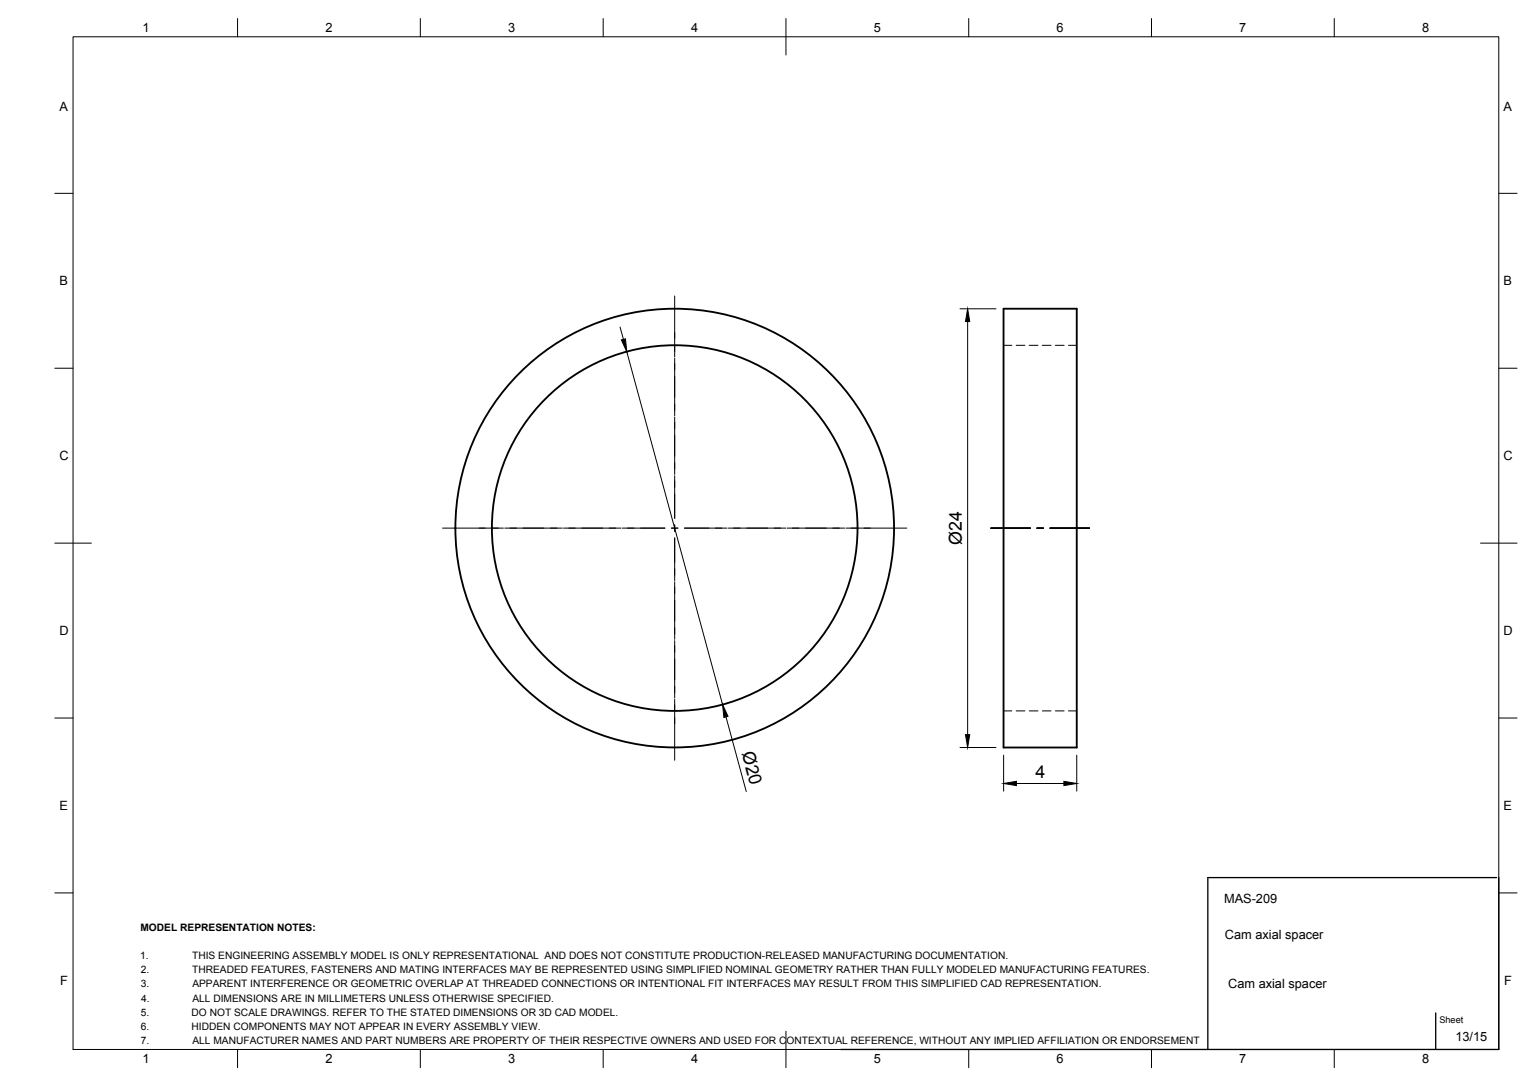
ISO-10303-21;
HEADER;
/* Generated by software containing ST-Developer
 * from STEP Tools, Inc. (www.steptools.com) 
 */

FILE_DESCRIPTION(
/* description */ ('Independent bearing-supported roller-ramp one-way clutch. Six logarit
hmic ramps with plain solid rollers, sprung guided plungers, native Co
il variants, removable shared keepers, rounded parallel key, shaft wit
h complete retaining lips, bronze journal/thrust support and bolted co
vers. Native rotor, roller planar/spin and plunger joints permit manua
l geometric engaged/released inspection. Automatic frictional torque s
witching/contact dynamics are not simulated; no capacity, hardness, fi
t, lubrication, speed, force or life rating. External input driver/cou
pling/anchors outside assembly.'),
/* implementation_level */ '2;1');

FILE_NAME(
/* name */ 'Cam axial spacer.step',
/* time_stamp */ '2026-11-08T07:04:38-08:00',
/* author */ (''),
/* organization */ (''),
/* preprocessor_version */ 'ST-DEVELOPER v20.2',
/* originating_system */ 'Autodesk Translation Framework v15.17.0.0',
/* authorisation */ '');

FILE_SCHEMA (('AUTOMOTIVE_DESIGN { 1 0 10303 214 3 1 1 }'));
ENDSEC;

DATA;
#10=MECHANICAL_DESIGN_GEOMETRIC_PRESENTATION_REPRESENTATION('',(#309),#99526);
#277=SHAPE_REPRESENTATION_RELATIONSHIP('SRR','None',#99634,#293);
#293=ADVANCED_BREP_SHAPE_REPRESENTATION('',(#325),#99519);
#309=STYLED_ITEM('',(#99721),#325);
#325=MANIFOLD_SOLID_BREP('Body1',#18279);
#432=FACE_BOUND('',#2670,.T.);
#433=FACE_BOUND('',#2672,.T.);
#581=PLANE('',#19610);
#582=PLANE('',#19611);
#1570=FACE_OUTER_BOUND('',#2667,.T.);
#1571=FACE_OUTER_BOUND('',#2668,.T.);
#1572=FACE_OUTER_BOUND('',#2669,.T.);
#1573=FACE_OUTER_BOUND('',#2671,.T.);
#2667=EDGE_LOOP('',(#16032,#16033,#16034,#16035));
#2668=EDGE_LOOP('',(#16036,#16037,#16038,#16039));
#2669=EDGE_LOOP('',(#16040));
#2670=EDGE_LOOP('',(#16041));
#2671=EDGE_LOOP('',(#16042));
#2672=EDGE_LOOP('',(#16043));
#3080=CIRCLE('',#19605,10.);
#3081=CIRCLE('',#19606,10.);
#3082=CIRCLE('',#19608,12.);
#3083=CIRCLE('',#19609,12.);
#5432=LINE('',#94869,#6336);
#5433=LINE('',#94875,#6337);
#6336=VECTOR('',#22887,10.);
#6337=VECTOR('',#22894,12.);
#8095=VERTEX_POINT('',#94866);
#8096=VERTEX_POINT('',#94868);
#8097=VERTEX_POINT('',#94872);
#8098=VERTEX_POINT('',#94874);
#10768=EDGE_CURVE('',#8095,#8095,#3080,.T.);
#10769=EDGE_CURVE('',#8095,#8096,#5432,.T.);
#10770=EDGE_CURVE('',#8096,#8096,#3081,.T.);
#10771=EDGE_CURVE('',#8097,#8097,#3082,.T.);
#10772=EDGE_CURVE('',#8097,#8098,#5433,.T.);
#10773=EDGE_CURVE('',#8098,#8098,#3083,.T.);
#16032=ORIENTED_EDGE('',*,*,#10768,.F.);
#16033=ORIENTED_EDGE('',*,*,#10769,.T.);
#16034=ORIENTED_EDGE('',*,*,#10770,.T.);
#16035=ORIENTED_EDGE('',*,*,#10769,.F.);
#16036=ORIENTED_EDGE('',*,*,#10771,.F.);
#16037=ORIENTED_EDGE('',*,*,#10772,.T.);
#16038=ORIENTED_EDGE('',*,*,#10773,.T.);
#16039=ORIENTED_EDGE('',*,*,#10772,.F.);
#16040=ORIENTED_EDGE('',*,*,#10771,.T.);
#16041=ORIENTED_EDGE('',*,*,#10768,.T.);
#16042=ORIENTED_EDGE('',*,*,#10773,.F.);
#16043=ORIENTED_EDGE('',*,*,#10770,.F.);
#17212=CYLINDRICAL_SURFACE('',#19604,10.);
#17213=CYLINDRICAL_SURFACE('',#19607,12.);
#18168=ADVANCED_FACE('',(#1570),#17212,.F.);
#18169=ADVANCED_FACE('',(#1571),#17213,.T.);
#18170=ADVANCED_FACE('',(#1572,#432),#581,.T.);
#18171=ADVANCED_FACE('',(#1573,#433),#582,.F.);
#18279=CLOSED_SHELL('',(#18168,#18169,#18170,#18171));
#19603=AXIS2_PLACEMENT_3D('',#94864,#22881,#22882);
#19604=AXIS2_PLACEMENT_3D('',#94865,#22883,#22884);
#19605=AXIS2_PLACEMENT_3D('',#94867,#22885,#22886);
#19606=AXIS2_PLACEMENT_3D('',#94870,#22888,#22889);
#19607=AXIS2_PLACEMENT_3D('',#94871,#22890,#22891);
#19608=AXIS2_PLACEMENT_3D('',#94873,#22892,#22893);
#19609=AXIS2_PLACEMENT_3D('',#94876,#22895,#22896);
#19610=AXIS2_PLACEMENT_3D('',#94877,#22897,#22898);
#19611=AXIS2_PLACEMENT_3D('',#94878,#22899,#22900);
#22881=DIRECTION('axis',(0.,0.,1.));
#22882=DIRECTION('refdir',(1.,0.,0.));
#22883=DIRECTION('center_axis',(0.,0.,1.));
#22884=DIRECTION('ref_axis',(1.,0.,0.));
#22885=DIRECTION('center_axis',(0.,0.,-1.));
#22886=DIRECTION('ref_axis',(1.,0.,0.));
#22887=DIRECTION('',(0.,0.,-1.));
#22888=DIRECTION('center_axis',(0.,0.,-1.));
#22889=DIRECTION('ref_axis',(1.,0.,0.));
#22890=DIRECTION('center_axis',(0.,0.,1.));
#22891=DIRECTION('ref_axis',(1.,0.,0.));
#22892=DIRECTION('center_axis',(0.,0.,1.));
#22893=DIRECTION('ref_axis',(1.,0.,0.));
#22894=DIRECTION('',(0.,0.,-1.));
#22895=DIRECTION('center_axis',(0.,0.,1.));
#22896=DIRECTION('ref_axis',(1.,0.,0.));
#22897=DIRECTION('center_axis',(0.,0.,1.));
#22898=DIRECTION('ref_axis',(1.,0.,0.));
#22899=DIRECTION('center_axis',(0.,0.,1.));
#22900=DIRECTION('ref_axis',(1.,0.,0.));
#94864=CARTESIAN_POINT('',(0.,0.,0.));
#94865=CARTESIAN_POINT('Origin',(0.,0.,0.));
#94866=CARTESIAN_POINT('',(-10.,-1.22464679914735E-15,4.));
#94867=CARTESIAN_POINT('Origin',(0.,0.,4.));
#94868=CARTESIAN_POINT('',(-10.,-1.22464679914735E-15,0.));
#94869=CARTESIAN_POINT('',(-10.,-1.22464679914735E-15,0.));
#94870=CARTESIAN_POINT('Origin',(0.,0.,0.));
#94871=CARTESIAN_POINT('Origin',(0.,0.,0.));
#94872=CARTESIAN_POINT('',(-12.,-1.46957615897682E-15,4.));
#94873=CARTESIAN_POINT('Origin',(0.,0.,4.));
#94874=CARTESIAN_POINT('',(-12.,-1.46957615897682E-15,0.));
#94875=CARTESIAN_POINT('',(-12.,-1.46957615897682E-15,0.));
#94876=CARTESIAN_POINT('Origin',(0.,0.,0.));
#94877=CARTESIAN_POINT('Origin',(0.,0.,4.));
#94878=CARTESIAN_POINT('Origin',(0.,0.,0.));
#99501=UNCERTAINTY_MEASURE_WITH_UNIT(LENGTH_MEASURE(0.01),#99527,
'DISTANCE_ACCURACY_VALUE',
'Maximum model space distance between geometric entities at asserted c
onnectivities');
#99508=UNCERTAINTY_MEASURE_WITH_UNIT(LENGTH_MEASURE(0.01),#99527,
'DISTANCE_ACCURACY_VALUE',
'Maximum model space distance between geometric entities at asserted c
onnectivities');
#99519=(
GEOMETRIC_REPRESENTATION_CONTEXT(3)
GLOBAL_UNCERTAINTY_ASSIGNED_CONTEXT((#99501))
GLOBAL_UNIT_ASSIGNED_CONTEXT((#99527,#99529,#99530))
REPRESENTATION_CONTEXT('','3D')
);
#99526=(
GEOMETRIC_REPRESENTATION_CONTEXT(3)
GLOBAL_UNCERTAINTY_ASSIGNED_CONTEXT((#99508))
GLOBAL_UNIT_ASSIGNED_CONTEXT((#99527,#99529,#99530))
REPRESENTATION_CONTEXT('','3D')
);
#99527=(
LENGTH_UNIT()
NAMED_UNIT(*)
SI_UNIT(.MILLI.,.METRE.)
);
#99529=(
NAMED_UNIT(*)
PLANE_ANGLE_UNIT()
SI_UNIT($,.RADIAN.)
);
#99530=(
NAMED_UNIT(*)
SI_UNIT($,.STERADIAN.)
SOLID_ANGLE_UNIT()
);
#99541=SHAPE_DEFINITION_REPRESENTATION(#99558,#99634);
#99558=PRODUCT_DEFINITION_SHAPE('',$,#99652);
#99634=SHAPE_REPRESENTATION('',(#19603),#99519);
#99641=PRODUCT_DEFINITION_CONTEXT('part definition',#99694,'design');
#99652=PRODUCT_DEFINITION('Cam axial spacer','Cam axial spacer',#99669,
#99641);
#99669=PRODUCT_DEFINITION_FORMATION('',$,#99706);
#99694=APPLICATION_CONTEXT(
'Core Data for Automotive Mechanical Design Process');
#99695=PRODUCT_CONTEXT('part definition',#99694,'mechanical');
#99706=PRODUCT('Cam axial spacer','Cam axial spacer',$,(#99695));
#99721=PRESENTATION_STYLE_ASSIGNMENT((#99734));
#99734=SURFACE_STYLE_USAGE(.BOTH.,#99747);
#99747=SURFACE_SIDE_STYLE('',(#99760));
#99760=SURFACE_STYLE_FILL_AREA(#99773);
#99773=FILL_AREA_STYLE('Spacer gray',(#99786));
#99786=FILL_AREA_STYLE_COLOUR('Spacer gray',#99799);
#99799=COLOUR_RGB('Spacer gray',0.576470588235294,0.615686274509804,0.666666666666667);
ENDSEC;
END-ISO-10303-21;
